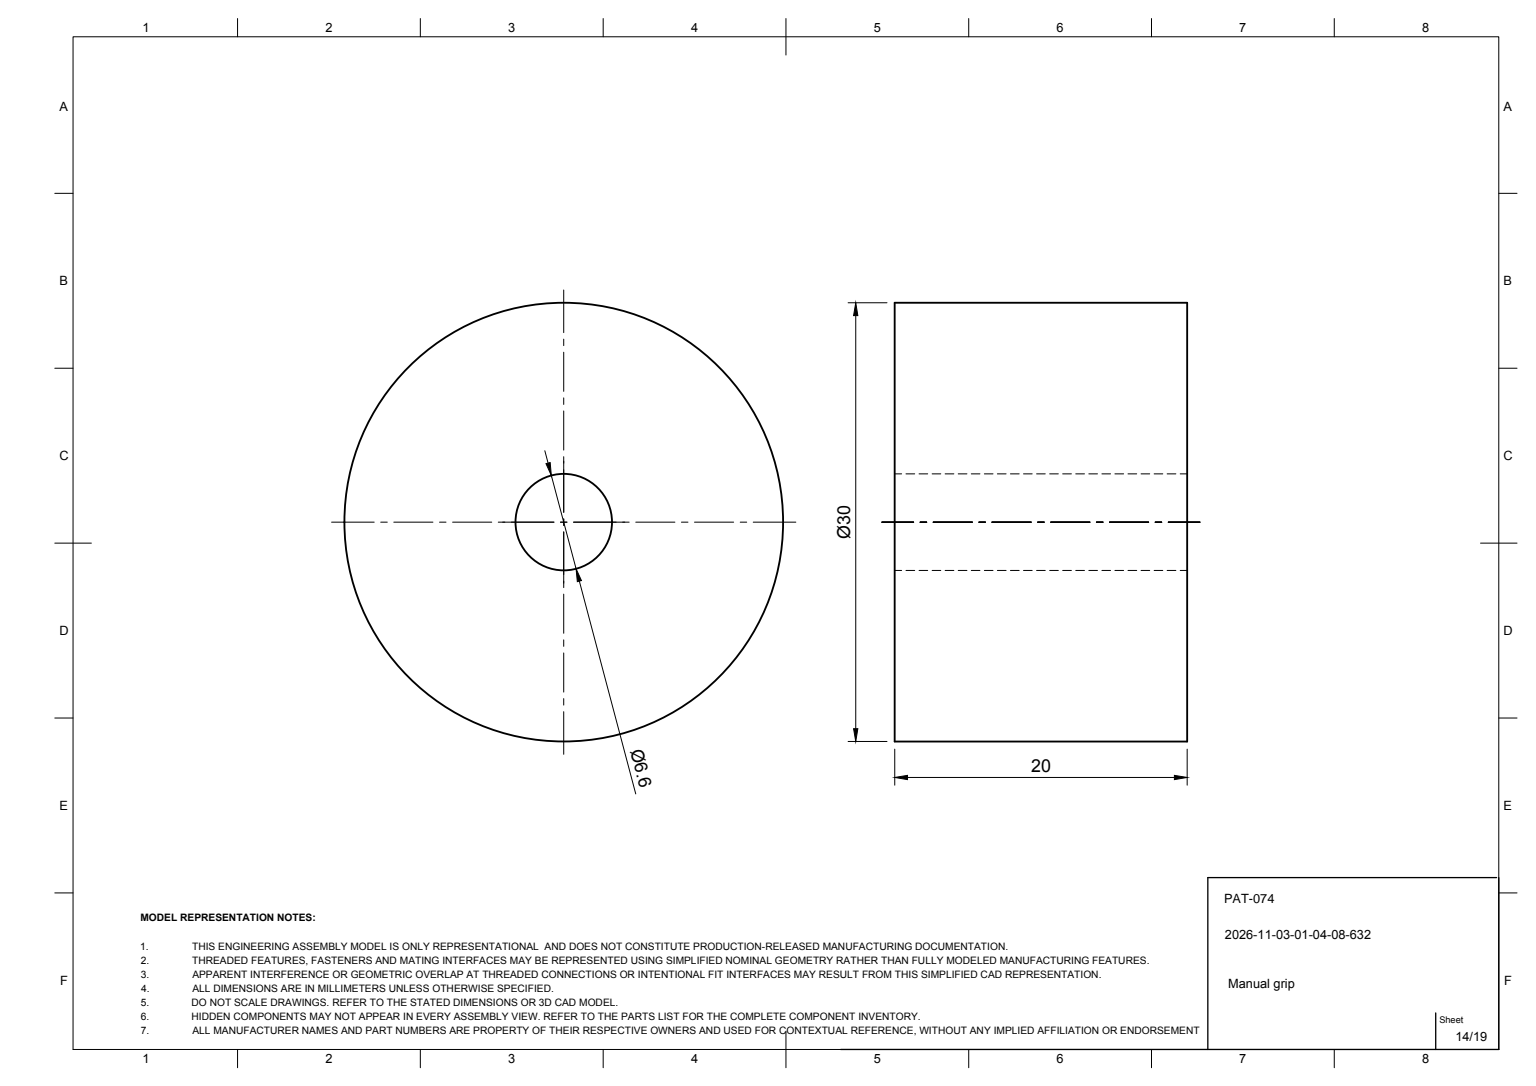
ISO-10303-21;
HEADER;
/* Generated by software containing ST-Developer
 * from STEP Tools, Inc. (www.steptools.com) 
 */

FILE_DESCRIPTION(
/* description */ ('Manual rail carriage with stops'),
/* implementation_level */ '2;1');

FILE_NAME(
/* name */ 'Manual grip.step',
/* time_stamp */ '2026-10-27T18:54:27-07:00',
/* author */ (''),
/* organization */ (''),
/* preprocessor_version */ 'ST-DEVELOPER v20.2',
/* originating_system */ 'Autodesk Translation Framework v15.17.0.0',
/* authorisation */ '');

FILE_SCHEMA (('AUTOMOTIVE_DESIGN { 1 0 10303 214 3 1 1 }'));
ENDSEC;

DATA;
#10=MECHANICAL_DESIGN_GEOMETRIC_PRESENTATION_REPRESENTATION('',(#286),#8499);
#250=SHAPE_REPRESENTATION_RELATIONSHIP('SRR','None',#8615,#268);
#268=ADVANCED_BREP_SHAPE_REPRESENTATION('',(#302),#8494);
#286=STYLED_ITEM('',(#8795),#302);
#302=MANIFOLD_SOLID_BREP('Body1',#4956);
#372=FACE_BOUND('',#1130,.T.);
#373=FACE_BOUND('',#1132,.T.);
#549=PLANE('',#5510);
#550=PLANE('',#5511);
#795=FACE_OUTER_BOUND('',#1127,.T.);
#796=FACE_OUTER_BOUND('',#1128,.T.);
#797=FACE_OUTER_BOUND('',#1129,.T.);
#798=FACE_OUTER_BOUND('',#1131,.T.);
#1127=EDGE_LOOP('',(#4456,#4457,#4458,#4459));
#1128=EDGE_LOOP('',(#4460,#4461,#4462,#4463));
#1129=EDGE_LOOP('',(#4464));
#1130=EDGE_LOOP('',(#4465));
#1131=EDGE_LOOP('',(#4466));
#1132=EDGE_LOOP('',(#4467));
#1627=LINE('',#8223,#2127);
#1628=LINE('',#8229,#2128);
#2127=VECTOR('',#6764,0.33);
#2128=VECTOR('',#6771,1.5);
#2283=CIRCLE('',#5505,0.33);
#2284=CIRCLE('',#5506,0.33);
#2285=CIRCLE('',#5508,1.5);
#2286=CIRCLE('',#5509,1.5);
#2675=VERTEX_POINT('',#8220);
#2676=VERTEX_POINT('',#8222);
#2677=VERTEX_POINT('',#8226);
#2678=VERTEX_POINT('',#8228);
#3276=EDGE_CURVE('',#2675,#2675,#2283,.T.);
#3277=EDGE_CURVE('',#2675,#2676,#1627,.T.);
#3278=EDGE_CURVE('',#2676,#2676,#2284,.T.);
#3279=EDGE_CURVE('',#2677,#2677,#2285,.T.);
#3280=EDGE_CURVE('',#2677,#2678,#1628,.T.);
#3281=EDGE_CURVE('',#2678,#2678,#2286,.T.);
#4456=ORIENTED_EDGE('',*,*,#3276,.F.);
#4457=ORIENTED_EDGE('',*,*,#3277,.T.);
#4458=ORIENTED_EDGE('',*,*,#3278,.T.);
#4459=ORIENTED_EDGE('',*,*,#3277,.F.);
#4460=ORIENTED_EDGE('',*,*,#3279,.F.);
#4461=ORIENTED_EDGE('',*,*,#3280,.T.);
#4462=ORIENTED_EDGE('',*,*,#3281,.T.);
#4463=ORIENTED_EDGE('',*,*,#3280,.F.);
#4464=ORIENTED_EDGE('',*,*,#3279,.T.);
#4465=ORIENTED_EDGE('',*,*,#3276,.T.);
#4466=ORIENTED_EDGE('',*,*,#3281,.F.);
#4467=ORIENTED_EDGE('',*,*,#3278,.F.);
#4666=CYLINDRICAL_SURFACE('',#5504,0.33);
#4667=CYLINDRICAL_SURFACE('',#5507,1.5);
#4894=ADVANCED_FACE('',(#795),#4666,.F.);
#4895=ADVANCED_FACE('',(#796),#4667,.T.);
#4896=ADVANCED_FACE('',(#797,#372),#549,.T.);
#4897=ADVANCED_FACE('',(#798,#373),#550,.F.);
#4956=CLOSED_SHELL('',(#4894,#4895,#4896,#4897));
#5503=AXIS2_PLACEMENT_3D('',#8218,#6758,#6759);
#5504=AXIS2_PLACEMENT_3D('',#8219,#6760,#6761);
#5505=AXIS2_PLACEMENT_3D('',#8221,#6762,#6763);
#5506=AXIS2_PLACEMENT_3D('',#8224,#6765,#6766);
#5507=AXIS2_PLACEMENT_3D('',#8225,#6767,#6768);
#5508=AXIS2_PLACEMENT_3D('',#8227,#6769,#6770);
#5509=AXIS2_PLACEMENT_3D('',#8230,#6772,#6773);
#5510=AXIS2_PLACEMENT_3D('',#8231,#6774,#6775);
#5511=AXIS2_PLACEMENT_3D('',#8232,#6776,#6777);
#6758=DIRECTION('axis',(0.,0.,1.));
#6759=DIRECTION('refdir',(1.,0.,0.));
#6760=DIRECTION('center_axis',(0.,0.,1.));
#6761=DIRECTION('ref_axis',(1.,0.,0.));
#6762=DIRECTION('center_axis',(0.,0.,-1.));
#6763=DIRECTION('ref_axis',(1.,0.,0.));
#6764=DIRECTION('',(0.,0.,-1.));
#6765=DIRECTION('center_axis',(0.,0.,-1.));
#6766=DIRECTION('ref_axis',(1.,0.,0.));
#6767=DIRECTION('center_axis',(0.,0.,1.));
#6768=DIRECTION('ref_axis',(1.,0.,0.));
#6769=DIRECTION('center_axis',(0.,0.,1.));
#6770=DIRECTION('ref_axis',(1.,0.,0.));
#6771=DIRECTION('',(0.,0.,-1.));
#6772=DIRECTION('center_axis',(0.,0.,1.));
#6773=DIRECTION('ref_axis',(1.,0.,0.));
#6774=DIRECTION('center_axis',(0.,0.,1.));
#6775=DIRECTION('ref_axis',(1.,0.,0.));
#6776=DIRECTION('center_axis',(0.,0.,1.));
#6777=DIRECTION('ref_axis',(1.,0.,0.));
#8218=CARTESIAN_POINT('',(0.,0.,0.));
#8219=CARTESIAN_POINT('Origin',(11.,0.,6.4));
#8220=CARTESIAN_POINT('',(10.67,-4.04133443718627E-17,8.4));
#8221=CARTESIAN_POINT('Origin',(11.,0.,8.4));
#8222=CARTESIAN_POINT('',(10.67,-4.04133443718627E-17,6.4));
#8223=CARTESIAN_POINT('',(10.67,-4.04133443718627E-17,6.4));
#8224=CARTESIAN_POINT('Origin',(11.,0.,6.4));
#8225=CARTESIAN_POINT('Origin',(11.,0.,6.4));
#8226=CARTESIAN_POINT('',(9.5,-1.83697019872103E-16,8.4));
#8227=CARTESIAN_POINT('Origin',(11.,0.,8.4));
#8228=CARTESIAN_POINT('',(9.5,-1.83697019872103E-16,6.4));
#8229=CARTESIAN_POINT('',(9.5,-1.83697019872103E-16,6.4));
#8230=CARTESIAN_POINT('Origin',(11.,0.,6.4));
#8231=CARTESIAN_POINT('Origin',(11.,0.,8.4));
#8232=CARTESIAN_POINT('Origin',(11.,0.,6.4));
#8471=UNCERTAINTY_MEASURE_WITH_UNIT(LENGTH_MEASURE(0.001),#8500,
'DISTANCE_ACCURACY_VALUE',
'Maximum model space distance between geometric entities at asserted c
onnectivities');
#8476=UNCERTAINTY_MEASURE_WITH_UNIT(LENGTH_MEASURE(0.001),#8500,
'DISTANCE_ACCURACY_VALUE',
'Maximum model space distance between geometric entities at asserted c
onnectivities');
#8494=(
GEOMETRIC_REPRESENTATION_CONTEXT(3)
GLOBAL_UNCERTAINTY_ASSIGNED_CONTEXT((#8471))
GLOBAL_UNIT_ASSIGNED_CONTEXT((#8500,#8502,#8503))
REPRESENTATION_CONTEXT('','3D')
);
#8499=(
GEOMETRIC_REPRESENTATION_CONTEXT(3)
GLOBAL_UNCERTAINTY_ASSIGNED_CONTEXT((#8476))
GLOBAL_UNIT_ASSIGNED_CONTEXT((#8500,#8502,#8503))
REPRESENTATION_CONTEXT('','3D')
);
#8500=(
LENGTH_UNIT()
NAMED_UNIT(*)
SI_UNIT(.CENTI.,.METRE.)
);
#8502=(
NAMED_UNIT(*)
PLANE_ANGLE_UNIT()
SI_UNIT($,.RADIAN.)
);
#8503=(
NAMED_UNIT(*)
SI_UNIT($,.STERADIAN.)
SOLID_ANGLE_UNIT()
);
#8521=SHAPE_DEFINITION_REPRESENTATION(#8546,#8615);
#8546=PRODUCT_DEFINITION_SHAPE('',$,#8638);
#8615=SHAPE_REPRESENTATION('',(#5503),#8494);
#8620=PRODUCT_DEFINITION_CONTEXT('part definition',#8688,'design');
#8638=PRODUCT_DEFINITION('Manual grip','Manual grip',#8660,#8620);
#8660=PRODUCT_DEFINITION_FORMATION('',$,#8707);
#8688=APPLICATION_CONTEXT(
'Core Data for Automotive Mechanical Design Process');
#8689=PRODUCT_CONTEXT('part definition',#8688,'mechanical');
#8707=PRODUCT('Manual grip','Manual grip','Manual grip',(#8689));
#8789=COLOUR_RGB('Black',0.12,0.14,0.17);
#8790=FILL_AREA_STYLE_COLOUR('',#8789);
#8791=FILL_AREA_STYLE('',(#8790));
#8792=SURFACE_STYLE_FILL_AREA(#8791);
#8793=SURFACE_SIDE_STYLE('',(#8792));
#8794=SURFACE_STYLE_USAGE(.BOTH.,#8793);
#8795=PRESENTATION_STYLE_ASSIGNMENT((#8794));
ENDSEC;
END-ISO-10303-21;
